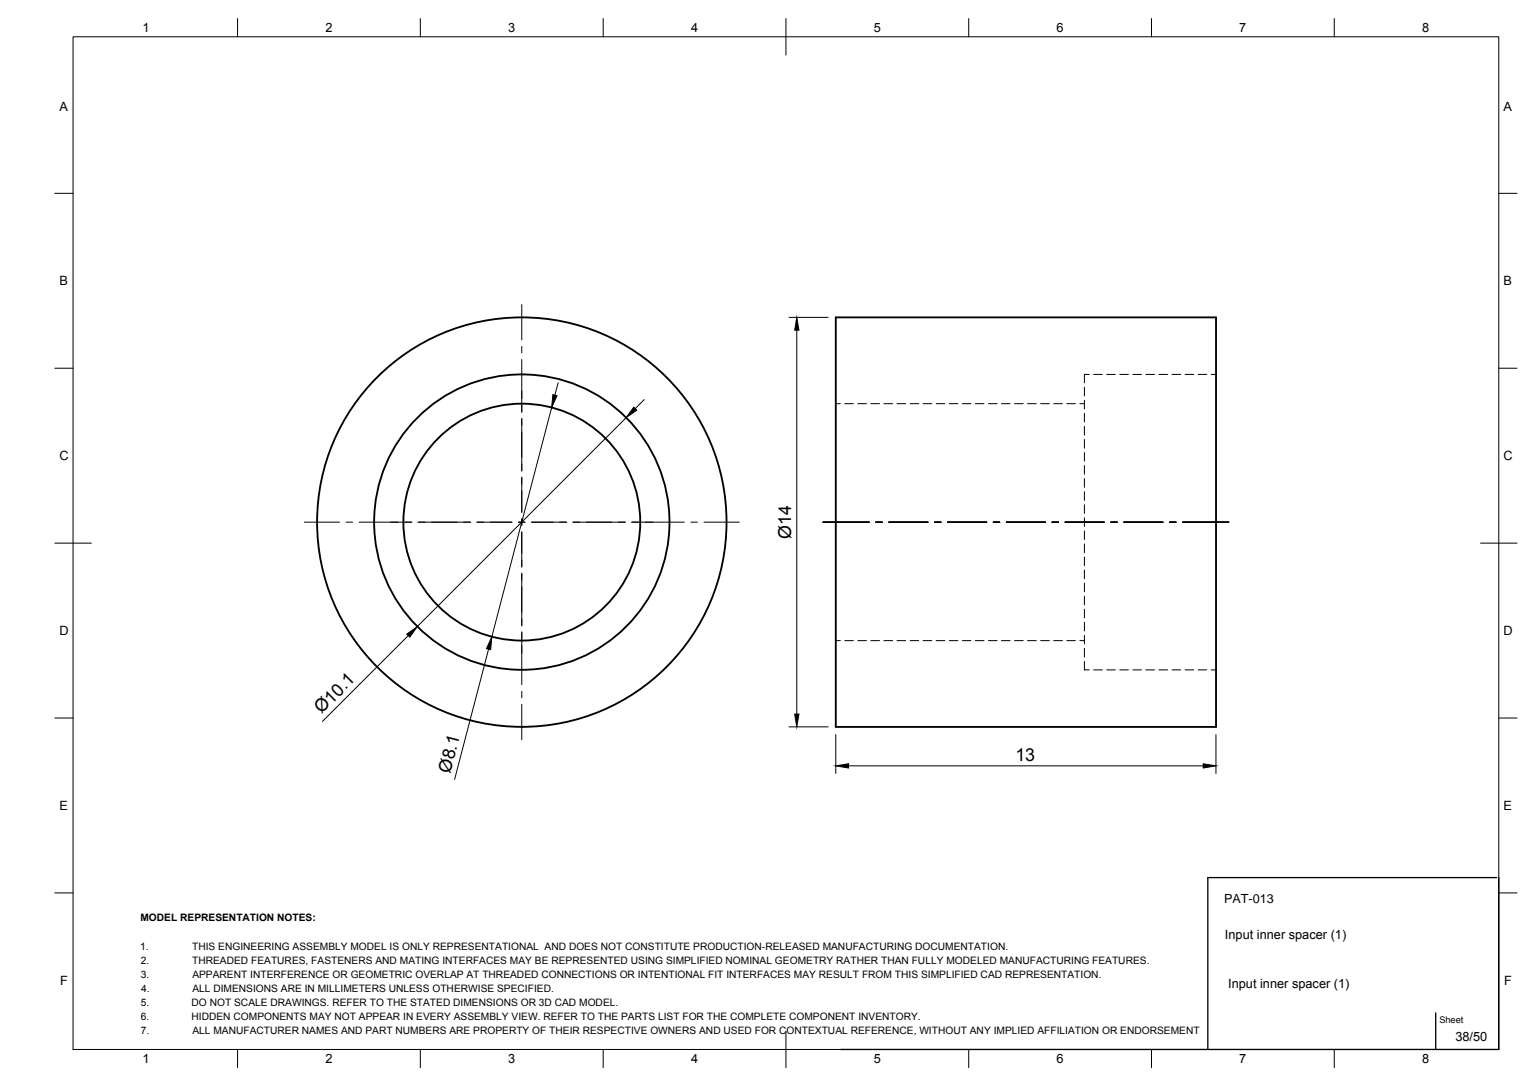
ISO-10303-21;
HEADER;
/* Generated by software containing ST-Developer
 * from STEP Tools, Inc. (www.steptools.com) 
 */

FILE_DESCRIPTION(
/* description */ ('Belt-driven linear axis on 2020 extrusion'),
/* implementation_level */ '2;1');

FILE_NAME(
/* name */ 'Input inner spacer (1).step',
/* time_stamp */ '2026-10-28T03:26:09-07:00',
/* author */ (''),
/* organization */ (''),
/* preprocessor_version */ 'ST-DEVELOPER v20.2',
/* originating_system */ 'Autodesk Translation Framework v15.17.0.0',
/* authorisation */ '');

FILE_SCHEMA (('AUTOMOTIVE_DESIGN { 1 0 10303 214 3 1 1 }'));
ENDSEC;

DATA;
#10=MECHANICAL_DESIGN_GEOMETRIC_PRESENTATION_REPRESENTATION('',(#650),#20096);
#548=SHAPE_REPRESENTATION_RELATIONSHIP('SRR','None',#20347,#594);
#594=ADVANCED_BREP_SHAPE_REPRESENTATION('',(#705),#20078);
#650=STYLED_ITEM('',(#20664),#705);
#705=MANIFOLD_SOLID_BREP('Body1',#10964);
#844=FACE_BOUND('',#2410,.T.);
#845=FACE_BOUND('',#2414,.T.);
#846=FACE_BOUND('',#2416,.T.);
#1133=PLANE('',#12281);
#1134=PLANE('',#12288);
#1135=PLANE('',#12289);
#1660=FACE_OUTER_BOUND('',#2408,.T.);
#1661=FACE_OUTER_BOUND('',#2409,.T.);
#1662=FACE_OUTER_BOUND('',#2411,.T.);
#1663=FACE_OUTER_BOUND('',#2412,.T.);
#1664=FACE_OUTER_BOUND('',#2413,.T.);
#1665=FACE_OUTER_BOUND('',#2415,.T.);
#2408=EDGE_LOOP('',(#9079,#9080,#9081,#9082));
#2409=EDGE_LOOP('',(#9083));
#2410=EDGE_LOOP('',(#9084));
#2411=EDGE_LOOP('',(#9085,#9086,#9087,#9088));
#2412=EDGE_LOOP('',(#9089,#9090,#9091,#9092));
#2413=EDGE_LOOP('',(#9093));
#2414=EDGE_LOOP('',(#9094));
#2415=EDGE_LOOP('',(#9095));
#2416=EDGE_LOOP('',(#9096));
#3223=LINE('',#18555,#4080);
#3224=LINE('',#18562,#4081);
#3225=LINE('',#18568,#4082);
#4080=VECTOR('',#14923,0.505000000000003);
#4081=VECTOR('',#14932,0.405000000000001);
#4082=VECTOR('',#14939,0.700000000000003);
#4714=CIRCLE('',#12279,0.505000000000003);
#4715=CIRCLE('',#12280,0.505000000000003);
#4716=CIRCLE('',#12282,0.405000000000001);
#4717=CIRCLE('',#12284,0.405000000000001);
#4718=CIRCLE('',#12286,0.700000000000003);
#4719=CIRCLE('',#12287,0.700000000000003);
#5509=VERTEX_POINT('',#18552);
#5510=VERTEX_POINT('',#18554);
#5511=VERTEX_POINT('',#18558);
#5512=VERTEX_POINT('',#18561);
#5513=VERTEX_POINT('',#18565);
#5514=VERTEX_POINT('',#18567);
#6754=EDGE_CURVE('',#5509,#5509,#4714,.T.);
#6755=EDGE_CURVE('',#5509,#5510,#3223,.T.);
#6756=EDGE_CURVE('',#5510,#5510,#4715,.T.);
#6757=EDGE_CURVE('',#5511,#5511,#4716,.T.);
#6758=EDGE_CURVE('',#5511,#5512,#3224,.T.);
#6759=EDGE_CURVE('',#5512,#5512,#4717,.T.);
#6760=EDGE_CURVE('',#5513,#5513,#4718,.T.);
#6761=EDGE_CURVE('',#5513,#5514,#3225,.T.);
#6762=EDGE_CURVE('',#5514,#5514,#4719,.T.);
#9079=ORIENTED_EDGE('',*,*,#6754,.F.);
#9080=ORIENTED_EDGE('',*,*,#6755,.T.);
#9081=ORIENTED_EDGE('',*,*,#6756,.F.);
#9082=ORIENTED_EDGE('',*,*,#6755,.F.);
#9083=ORIENTED_EDGE('',*,*,#6754,.T.);
#9084=ORIENTED_EDGE('',*,*,#6757,.F.);
#9085=ORIENTED_EDGE('',*,*,#6757,.T.);
#9086=ORIENTED_EDGE('',*,*,#6758,.T.);
#9087=ORIENTED_EDGE('',*,*,#6759,.T.);
#9088=ORIENTED_EDGE('',*,*,#6758,.F.);
#9089=ORIENTED_EDGE('',*,*,#6760,.F.);
#9090=ORIENTED_EDGE('',*,*,#6761,.T.);
#9091=ORIENTED_EDGE('',*,*,#6762,.T.);
#9092=ORIENTED_EDGE('',*,*,#6761,.F.);
#9093=ORIENTED_EDGE('',*,*,#6760,.T.);
#9094=ORIENTED_EDGE('',*,*,#6756,.T.);
#9095=ORIENTED_EDGE('',*,*,#6762,.F.);
#9096=ORIENTED_EDGE('',*,*,#6759,.F.);
#10218=CYLINDRICAL_SURFACE('',#12278,0.505000000000003);
#10219=CYLINDRICAL_SURFACE('',#12283,0.405000000000001);
#10220=CYLINDRICAL_SURFACE('',#12285,0.700000000000003);
#10711=ADVANCED_FACE('',(#1660),#10218,.F.);
#10712=ADVANCED_FACE('',(#1661,#844),#1133,.T.);
#10713=ADVANCED_FACE('',(#1662),#10219,.F.);
#10714=ADVANCED_FACE('',(#1663),#10220,.T.);
#10715=ADVANCED_FACE('',(#1664,#845),#1134,.T.);
#10716=ADVANCED_FACE('',(#1665,#846),#1135,.F.);
#10964=CLOSED_SHELL('',(#10711,#10712,#10713,#10714,#10715,#10716));
#12277=AXIS2_PLACEMENT_3D('',#18550,#14917,#14918);
#12278=AXIS2_PLACEMENT_3D('',#18551,#14919,#14920);
#12279=AXIS2_PLACEMENT_3D('',#18553,#14921,#14922);
#12280=AXIS2_PLACEMENT_3D('',#18556,#14924,#14925);
#12281=AXIS2_PLACEMENT_3D('',#18557,#14926,#14927);
#12282=AXIS2_PLACEMENT_3D('',#18559,#14928,#14929);
#12283=AXIS2_PLACEMENT_3D('',#18560,#14930,#14931);
#12284=AXIS2_PLACEMENT_3D('',#18563,#14933,#14934);
#12285=AXIS2_PLACEMENT_3D('',#18564,#14935,#14936);
#12286=AXIS2_PLACEMENT_3D('',#18566,#14937,#14938);
#12287=AXIS2_PLACEMENT_3D('',#18569,#14940,#14941);
#12288=AXIS2_PLACEMENT_3D('',#18570,#14942,#14943);
#12289=AXIS2_PLACEMENT_3D('',#18571,#14944,#14945);
#14917=DIRECTION('axis',(0.,0.,1.));
#14918=DIRECTION('refdir',(1.,0.,0.));
#14919=DIRECTION('center_axis',(0.,1.,0.));
#14920=DIRECTION('ref_axis',(1.,0.,0.));
#14921=DIRECTION('center_axis',(0.,1.,0.));
#14922=DIRECTION('ref_axis',(1.,0.,0.));
#14923=DIRECTION('',(0.,1.,0.));
#14924=DIRECTION('center_axis',(0.,-1.,0.));
#14925=DIRECTION('ref_axis',(1.,0.,0.));
#14926=DIRECTION('center_axis',(0.,1.,0.));
#14927=DIRECTION('ref_axis',(1.,0.,0.));
#14928=DIRECTION('center_axis',(0.,1.,0.));
#14929=DIRECTION('ref_axis',(1.,0.,0.));
#14930=DIRECTION('center_axis',(0.,1.,0.));
#14931=DIRECTION('ref_axis',(1.,0.,0.));
#14932=DIRECTION('',(0.,-1.,0.));
#14933=DIRECTION('center_axis',(0.,-1.,0.));
#14934=DIRECTION('ref_axis',(1.,0.,0.));
#14935=DIRECTION('center_axis',(0.,1.,0.));
#14936=DIRECTION('ref_axis',(1.,0.,0.));
#14937=DIRECTION('center_axis',(0.,1.,0.));
#14938=DIRECTION('ref_axis',(1.,0.,0.));
#14939=DIRECTION('',(0.,-1.,0.));
#14940=DIRECTION('center_axis',(0.,1.,0.));
#14941=DIRECTION('ref_axis',(1.,0.,0.));
#14942=DIRECTION('center_axis',(0.,1.,0.));
#14943=DIRECTION('ref_axis',(1.,0.,0.));
#14944=DIRECTION('center_axis',(0.,1.,0.));
#14945=DIRECTION('ref_axis',(1.,0.,0.));
#18550=CARTESIAN_POINT('',(0.,0.,0.));
#18551=CARTESIAN_POINT('Origin',(32.,-1.8,7.));
#18552=CARTESIAN_POINT('',(31.495,-1.8,7.));
#18553=CARTESIAN_POINT('Origin',(32.,-1.8,7.));
#18554=CARTESIAN_POINT('',(31.495,-1.35,7.));
#18555=CARTESIAN_POINT('',(31.495,-1.8,7.));
#18556=CARTESIAN_POINT('Origin',(32.,-1.35,7.));
#18557=CARTESIAN_POINT('Origin',(32.,-1.8,7.));
#18558=CARTESIAN_POINT('',(31.595,-1.8,7.));
#18559=CARTESIAN_POINT('Origin',(32.,-1.8,7.));
#18560=CARTESIAN_POINT('Origin',(32.,-2.65,7.));
#18561=CARTESIAN_POINT('',(31.595,-2.65,7.));
#18562=CARTESIAN_POINT('',(31.595,-2.65,7.));
#18563=CARTESIAN_POINT('Origin',(32.,-2.65,7.));
#18564=CARTESIAN_POINT('Origin',(32.,-2.65,7.));
#18565=CARTESIAN_POINT('',(31.3,-1.35,7.));
#18566=CARTESIAN_POINT('Origin',(32.,-1.35,7.));
#18567=CARTESIAN_POINT('',(31.3,-2.65,7.));
#18568=CARTESIAN_POINT('',(31.3,-2.65,7.));
#18569=CARTESIAN_POINT('Origin',(32.,-2.65,7.));
#18570=CARTESIAN_POINT('Origin',(32.,-1.35,7.));
#18571=CARTESIAN_POINT('Origin',(32.,-2.65,7.));
#20024=UNCERTAINTY_MEASURE_WITH_UNIT(LENGTH_MEASURE(0.001),#20097,
'DISTANCE_ACCURACY_VALUE',
'Maximum model space distance between geometric entities at asserted c
onnectivities');
#20042=UNCERTAINTY_MEASURE_WITH_UNIT(LENGTH_MEASURE(0.001),#20097,
'DISTANCE_ACCURACY_VALUE',
'Maximum model space distance between geometric entities at asserted c
onnectivities');
#20078=(
GEOMETRIC_REPRESENTATION_CONTEXT(3)
GLOBAL_UNCERTAINTY_ASSIGNED_CONTEXT((#20024))
GLOBAL_UNIT_ASSIGNED_CONTEXT((#20097,#20099,#20100))
REPRESENTATION_CONTEXT('','3D')
);
#20096=(
GEOMETRIC_REPRESENTATION_CONTEXT(3)
GLOBAL_UNCERTAINTY_ASSIGNED_CONTEXT((#20042))
GLOBAL_UNIT_ASSIGNED_CONTEXT((#20097,#20099,#20100))
REPRESENTATION_CONTEXT('','3D')
);
#20097=(
LENGTH_UNIT()
NAMED_UNIT(*)
SI_UNIT(.CENTI.,.METRE.)
);
#20099=(
NAMED_UNIT(*)
PLANE_ANGLE_UNIT()
SI_UNIT($,.RADIAN.)
);
#20100=(
NAMED_UNIT(*)
SI_UNIT($,.STERADIAN.)
SOLID_ANGLE_UNIT()
);
#20136=SHAPE_DEFINITION_REPRESENTATION(#20194,#20347);
#20194=PRODUCT_DEFINITION_SHAPE('',$,#20401);
#20347=SHAPE_REPRESENTATION('',(#12277),#20078);
#20365=PRODUCT_DEFINITION_CONTEXT('part definition',#20526,'design');
#20401=PRODUCT_DEFINITION('Input inner spacer (1)',
'Input inner spacer (1)',#20454,#20365);
#20454=PRODUCT_DEFINITION_FORMATION('',$,#20563);
#20526=APPLICATION_CONTEXT(
'Core Data for Automotive Mechanical Design Process');
#20527=PRODUCT_CONTEXT('part definition',#20526,'mechanical');
#20563=PRODUCT('Input inner spacer (1)','Input inner spacer (1)',
'Input inner spacer (1)',(#20527));
#20658=COLOUR_RGB('Off White',0.89,0.88,0.83);
#20659=FILL_AREA_STYLE_COLOUR('',#20658);
#20660=FILL_AREA_STYLE('',(#20659));
#20661=SURFACE_STYLE_FILL_AREA(#20660);
#20662=SURFACE_SIDE_STYLE('',(#20661));
#20663=SURFACE_STYLE_USAGE(.BOTH.,#20662);
#20664=PRESENTATION_STYLE_ASSIGNMENT((#20663));
ENDSEC;
END-ISO-10303-21;
